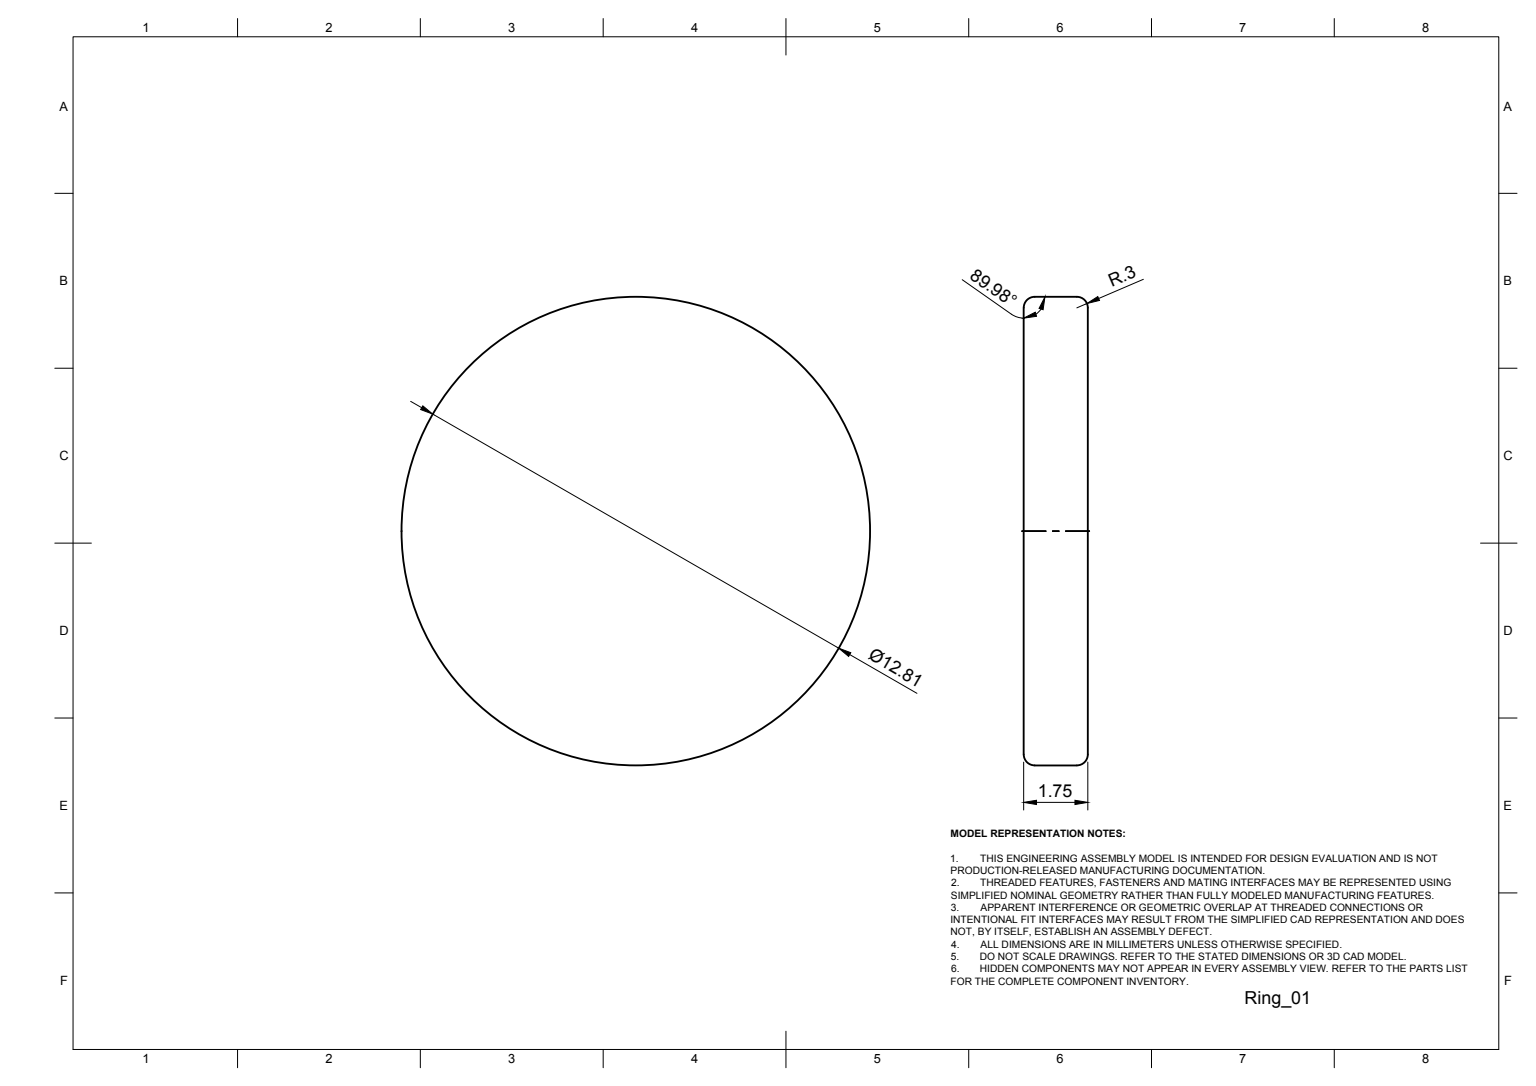
ISO-10303-21;
HEADER;
/* Generated by software containing ST-Developer
 * from STEP Tools, Inc. (www.steptools.com) 
 */

FILE_DESCRIPTION(
/* description */ (''),
/* implementation_level */ '2;1');

FILE_NAME(
/* name */ 'Ring_01.step',
/* time_stamp */ '2026-10-06T13:05:37-07:00',
/* author */ (''),
/* organization */ (''),
/* preprocessor_version */ 'ST-DEVELOPER v20.2',
/* originating_system */ 'Autodesk Translation Framework v15.15.0.0',
/* authorisation */ '');

FILE_SCHEMA (('AUTOMOTIVE_DESIGN { 1 0 10303 214 3 1 1 }'));
ENDSEC;

DATA;
#10=MECHANICAL_DESIGN_GEOMETRIC_PRESENTATION_REPRESENTATION('',(#141),#28055);
#112=TOROIDAL_SURFACE('',#4003,6.1074958342087,0.3);
#113=TOROIDAL_SURFACE('',#4010,6.1071549018742,0.3);
#121=SHAPE_REPRESENTATION_RELATIONSHIP('SRR','None',#28098,#131);
#131=ADVANCED_BREP_SHAPE_REPRESENTATION('',(#151),#28050);
#141=STYLED_ITEM('',(#28153),#151);
#151=MANIFOLD_SOLID_BREP('Body1',#3682);
#170=CONICAL_SURFACE('',#4007,6.40732538114918,0.000295609290232334);
#235=PLANE('',#4009);
#236=PLANE('',#4013);
#349=CIRCLE('',#4004,6.1074958342087);
#350=CIRCLE('',#4005,0.3);
#351=CIRCLE('',#4006,6.40749582110097);
#352=CIRCLE('',#4008,6.40715488876647);
#353=CIRCLE('',#4011,0.3);
#354=CIRCLE('',#4012,6.1071549018742);
#490=FACE_OUTER_BOUND('',#719,.T.);
#491=FACE_OUTER_BOUND('',#720,.T.);
#492=FACE_OUTER_BOUND('',#721,.T.);
#493=FACE_OUTER_BOUND('',#722,.T.);
#494=FACE_OUTER_BOUND('',#723,.T.);
#719=EDGE_LOOP('',(#2914,#2915,#2916,#2917));
#720=EDGE_LOOP('',(#2918,#2919,#2920,#2921));
#721=EDGE_LOOP('',(#2922));
#722=EDGE_LOOP('',(#2923,#2924,#2925,#2926));
#723=EDGE_LOOP('',(#2927));
#893=LINE('',#22145,#1051);
#1051=VECTOR('',#4602,6.40732538114918);
#1610=VERTEX_POINT('',#22138);
#1611=VERTEX_POINT('',#22140);
#1612=VERTEX_POINT('',#22144);
#1613=VERTEX_POINT('',#22149);
#2070=EDGE_CURVE('',#1610,#1610,#349,.T.);
#2071=EDGE_CURVE('',#1610,#1611,#350,.T.);
#2072=EDGE_CURVE('',#1611,#1611,#351,.T.);
#2073=EDGE_CURVE('',#1611,#1612,#893,.T.);
#2074=EDGE_CURVE('',#1612,#1612,#352,.T.);
#2075=EDGE_CURVE('',#1612,#1613,#353,.T.);
#2076=EDGE_CURVE('',#1613,#1613,#354,.T.);
#2914=ORIENTED_EDGE('',*,*,#2070,.T.);
#2915=ORIENTED_EDGE('',*,*,#2071,.T.);
#2916=ORIENTED_EDGE('',*,*,#2072,.T.);
#2917=ORIENTED_EDGE('',*,*,#2071,.F.);
#2918=ORIENTED_EDGE('',*,*,#2072,.F.);
#2919=ORIENTED_EDGE('',*,*,#2073,.T.);
#2920=ORIENTED_EDGE('',*,*,#2074,.F.);
#2921=ORIENTED_EDGE('',*,*,#2073,.F.);
#2922=ORIENTED_EDGE('',*,*,#2070,.F.);
#2923=ORIENTED_EDGE('',*,*,#2074,.T.);
#2924=ORIENTED_EDGE('',*,*,#2075,.T.);
#2925=ORIENTED_EDGE('',*,*,#2076,.T.);
#2926=ORIENTED_EDGE('',*,*,#2075,.F.);
#2927=ORIENTED_EDGE('',*,*,#2076,.F.);
#3582=ADVANCED_FACE('',(#490),#112,.T.);
#3583=ADVANCED_FACE('',(#491),#170,.T.);
#3584=ADVANCED_FACE('',(#492),#235,.T.);
#3585=ADVANCED_FACE('',(#493),#113,.T.);
#3586=ADVANCED_FACE('',(#494),#236,.T.);
#3682=CLOSED_SHELL('',(#3582,#3583,#3584,#3585,#3586));
#4002=AXIS2_PLACEMENT_3D('',#22136,#4590,#4591);
#4003=AXIS2_PLACEMENT_3D('',#22137,#4592,#4593);
#4004=AXIS2_PLACEMENT_3D('',#22139,#4594,#4595);
#4005=AXIS2_PLACEMENT_3D('',#22141,#4596,#4597);
#4006=AXIS2_PLACEMENT_3D('',#22142,#4598,#4599);
#4007=AXIS2_PLACEMENT_3D('',#22143,#4600,#4601);
#4008=AXIS2_PLACEMENT_3D('',#22146,#4603,#4604);
#4009=AXIS2_PLACEMENT_3D('',#22147,#4605,#4606);
#4010=AXIS2_PLACEMENT_3D('',#22148,#4607,#4608);
#4011=AXIS2_PLACEMENT_3D('',#22150,#4609,#4610);
#4012=AXIS2_PLACEMENT_3D('',#22151,#4611,#4612);
#4013=AXIS2_PLACEMENT_3D('',#22152,#4613,#4614);
#4590=DIRECTION('axis',(0.,0.,1.));
#4591=DIRECTION('refdir',(1.,0.,0.));
#4592=DIRECTION('center_axis',(1.,0.,0.));
#4593=DIRECTION('ref_axis',(0.,0.,-1.));
#4594=DIRECTION('center_axis',(-1.,0.,0.));
#4595=DIRECTION('ref_axis',(0.,1.22464679914735E-16,1.));
#4596=DIRECTION('center_axis',(0.,-1.,-1.22464679914735E-16));
#4597=DIRECTION('ref_axis',(0.,-1.22464679914735E-16,1.));
#4598=DIRECTION('center_axis',(1.,0.,0.));
#4599=DIRECTION('ref_axis',(0.,0.,1.));
#4600=DIRECTION('center_axis',(1.,0.,0.));
#4601=DIRECTION('ref_axis',(0.,0.,-1.));
#4602=DIRECTION('',(-0.999999956307574,3.62016965808782E-20,-0.000295609285927038));
#4603=DIRECTION('center_axis',(-1.,0.,0.));
#4604=DIRECTION('ref_axis',(0.,0.,1.));
#4605=DIRECTION('center_axis',(1.,0.,0.));
#4606=DIRECTION('ref_axis',(0.,0.,-1.));
#4607=DIRECTION('center_axis',(1.,0.,0.));
#4608=DIRECTION('ref_axis',(0.,0.,-1.));
#4609=DIRECTION('center_axis',(0.,-1.,-1.22464679914735E-16));
#4610=DIRECTION('ref_axis',(0.,-1.22464679914735E-16,1.));
#4611=DIRECTION('center_axis',(1.,0.,0.));
#4612=DIRECTION('ref_axis',(0.,1.22464679914735E-16,1.));
#4613=DIRECTION('center_axis',(-1.,0.,0.));
#4614=DIRECTION('ref_axis',(0.,0.,1.));
#22136=CARTESIAN_POINT('',(0.,0.,0.));
#22137=CARTESIAN_POINT('Origin',(24.2263990006525,0.,0.));
#22138=CARTESIAN_POINT('',(24.5263990006525,-7.47952522416948E-16,6.1074958342087));
#22139=CARTESIAN_POINT('Origin',(24.5263990006525,0.,0.));
#22140=CARTESIAN_POINT('',(24.2263103178667,-7.84691924786135E-16,6.40749582110097));
#22141=CARTESIAN_POINT('Origin',(24.2263990006525,-7.47952522416948E-16,
6.1074958342087));
#22142=CARTESIAN_POINT('Origin',(24.2263103178667,-7.84691924786135E-16,
0.));
#22143=CARTESIAN_POINT('Origin',(23.6497386319918,0.,0.));
#22144=CARTESIAN_POINT('',(23.0729895805454,-7.84650172616918E-16,6.40715488876647));
#22145=CARTESIAN_POINT('',(23.6497386319918,-7.84671051911994E-16,6.40732538114918));
#22146=CARTESIAN_POINT('Origin',(23.0729895805454,-7.84650172616918E-16,
0.));
#22147=CARTESIAN_POINT('Origin',(24.5263990006525,0.,0.));
#22148=CARTESIAN_POINT('Origin',(23.0730782633312,0.,0.));
#22149=CARTESIAN_POINT('',(22.7730782633312,-7.47910770247731E-16,6.1071549018742));
#22150=CARTESIAN_POINT('Origin',(23.0730782633312,-7.47910770247731E-16,
6.1071549018742));
#22151=CARTESIAN_POINT('Origin',(22.7730782633312,0.,0.));
#22152=CARTESIAN_POINT('Origin',(22.7730782633312,0.,-6.40706623219228));
#28038=UNCERTAINTY_MEASURE_WITH_UNIT(LENGTH_MEASURE(0.01),#28056,
'DISTANCE_ACCURACY_VALUE',
'Maximum model space distance between geometric entities at asserted c
onnectivities');
#28043=UNCERTAINTY_MEASURE_WITH_UNIT(LENGTH_MEASURE(0.01),#28056,
'DISTANCE_ACCURACY_VALUE',
'Maximum model space distance between geometric entities at asserted c
onnectivities');
#28050=(
GEOMETRIC_REPRESENTATION_CONTEXT(3)
GLOBAL_UNCERTAINTY_ASSIGNED_CONTEXT((#28038))
GLOBAL_UNIT_ASSIGNED_CONTEXT((#28056,#28058,#28059))
REPRESENTATION_CONTEXT('','3D')
);
#28055=(
GEOMETRIC_REPRESENTATION_CONTEXT(3)
GLOBAL_UNCERTAINTY_ASSIGNED_CONTEXT((#28043))
GLOBAL_UNIT_ASSIGNED_CONTEXT((#28056,#28058,#28059))
REPRESENTATION_CONTEXT('','3D')
);
#28056=(
LENGTH_UNIT()
NAMED_UNIT(*)
SI_UNIT(.MILLI.,.METRE.)
);
#28058=(
NAMED_UNIT(*)
PLANE_ANGLE_UNIT()
SI_UNIT($,.RADIAN.)
);
#28059=(
NAMED_UNIT(*)
SI_UNIT($,.STERADIAN.)
SOLID_ANGLE_UNIT()
);
#28066=SHAPE_DEFINITION_REPRESENTATION(#28077,#28098);
#28077=PRODUCT_DEFINITION_SHAPE('',$,#28110);
#28098=SHAPE_REPRESENTATION('',(#4002),#28050);
#28103=PRODUCT_DEFINITION_CONTEXT('part definition',#28138,'design');
#28110=PRODUCT_DEFINITION('Ring_01','Ring_01',#28121,#28103);
#28121=PRODUCT_DEFINITION_FORMATION('',$,#28146);
#28138=APPLICATION_CONTEXT(
'Core Data for Automotive Mechanical Design Process');
#28139=PRODUCT_CONTEXT('part definition',#28138,'mechanical');
#28146=PRODUCT('Ring_01','Ring_01',$,(#28139));
#28153=PRESENTATION_STYLE_ASSIGNMENT((#28156));
#28156=SURFACE_STYLE_USAGE(.BOTH.,#28159);
#28159=SURFACE_SIDE_STYLE('',(#28162));
#28162=SURFACE_STYLE_FILL_AREA(#28165);
#28165=FILL_AREA_STYLE('Opaque(39,39,39)',(#28168));
#28168=FILL_AREA_STYLE_COLOUR('Opaque(39,39,39)',#28171);
#28171=COLOUR_RGB('Opaque(39,39,39)', 0.08235294, 0.09019608, 0.10196078);
ENDSEC;
END-ISO-10303-21;
